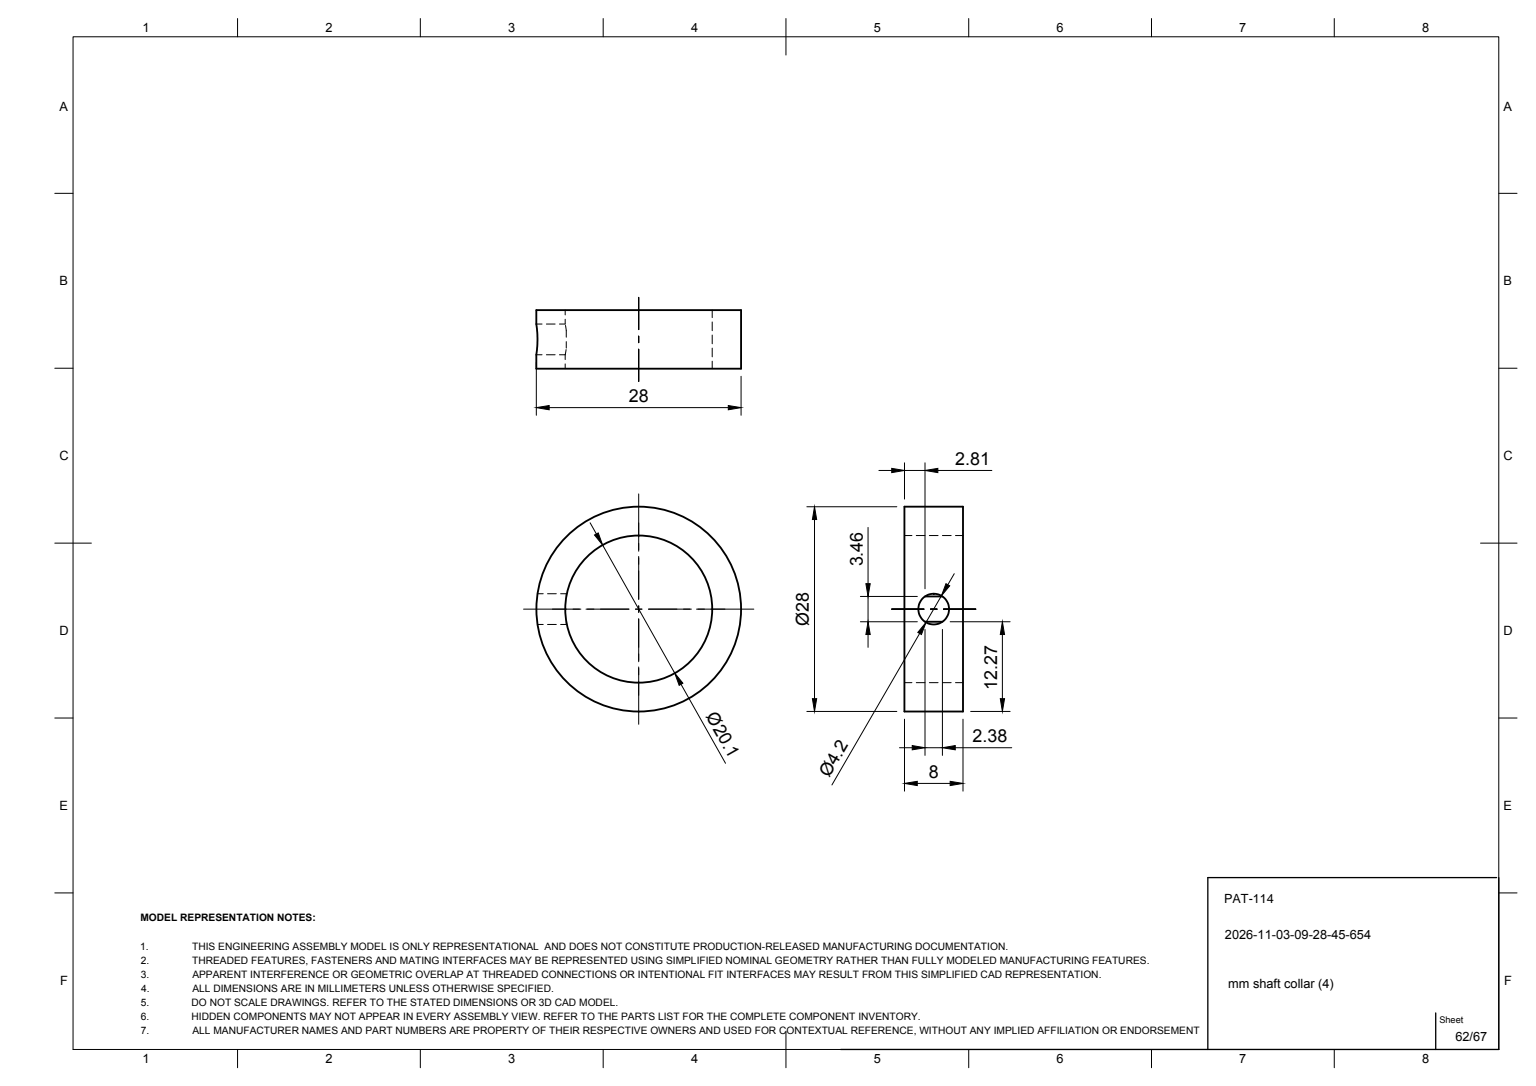
ISO-10303-21;
HEADER;
/* Generated by software containing ST-Developer
 * from STEP Tools, Inc. (www.steptools.com) 
 */

FILE_DESCRIPTION(
/* description */ ('Two-stage gear reducer in split housing'),
/* implementation_level */ '2;1');

FILE_NAME(
/* name */ 'mm shaft collar (4).step',
/* time_stamp */ '2026-10-28T03:22:31-07:00',
/* author */ (''),
/* organization */ (''),
/* preprocessor_version */ 'ST-DEVELOPER v20.2',
/* originating_system */ 'Autodesk Translation Framework v15.17.0.0',
/* authorisation */ '');

FILE_SCHEMA (('AUTOMOTIVE_DESIGN { 1 0 10303 214 3 1 1 }'));
ENDSEC;

DATA;
#10=MECHANICAL_DESIGN_GEOMETRIC_PRESENTATION_REPRESENTATION('',(#1296),#73366);
#979=B_SPLINE_CURVE_WITH_KNOTS('',3,(#49298,#49299,#49300,#49301,#49302,
#49303,#49304,#49305,#49306,#49307,#49308,#49309,#49310,#49311),
 .UNSPECIFIED.,.F.,.F.,(4,2,2,2,2,2,4),(0.756005737987022,0.79356882756465,
0.872922520054205,0.95227621254376,1.03162990503331,1.11098359752287,1.14854668710049),
 .UNSPECIFIED.);
#980=B_SPLINE_CURVE_WITH_KNOTS('',3,(#49317,#49318,#49319,#49320,#49321,
#49322,#49323,#49324,#49325,#49326,#49327,#49328,#49329,#49330,#49331,#49332,
#49333,#49334),.UNSPECIFIED.,.F.,.F.,(4,2,2,2,2,2,2,2,4),(0.,0.0792334805614376,
0.158466961122875,0.237699060165218,0.316931159207561,0.396163258249904,
0.475395357292247,0.554628837853685,0.633862318415122),.UNSPECIFIED.);
#981=B_SPLINE_CURVE_WITH_KNOTS('',3,(#49335,#49336,#49337,#49338,#49339,
#49340,#49341,#49342,#49343,#49344,#49345,#49346,#49347,#49348,#49349,#49350,
#49351,#49352),.UNSPECIFIED.,.F.,.F.,(4,2,2,2,2,2,2,2,4),(0.633862318415122,
0.71309579897656,0.792329279537998,0.871561378580341,0.950793477622684,
1.03002557666503,1.10925767570737,1.18849115626881,1.26772463683024),
 .UNSPECIFIED.);
#982=B_SPLINE_CURVE_WITH_KNOTS('',3,(#49355,#49356,#49357,#49358,#49359,
#49360,#49361,#49362,#49363,#49364,#49365,#49366,#49367,#49368),
 .UNSPECIFIED.,.F.,.F.,(4,2,2,2,2,2,4),(0.121154929624522,0.158718019202143,
0.238071711691698,0.317425404181253,0.396779096670808,0.476132789160363,
0.513695878737986),.UNSPECIFIED.);
#1169=SHAPE_REPRESENTATION_RELATIONSHIP('SRR','None',#73661,#1225);
#1225=ADVANCED_BREP_SHAPE_REPRESENTATION('',(#1365),#73357);
#1296=STYLED_ITEM('',(#73988),#1365);
#1365=MANIFOLD_SOLID_BREP('Body1',#16186);
#1582=FACE_BOUND('',#3820,.T.);
#1583=FACE_BOUND('',#3822,.T.);
#1584=FACE_BOUND('',#3824,.T.);
#1585=FACE_BOUND('',#3826,.T.);
#1921=PLANE('',#18152);
#1922=PLANE('',#18157);
#1923=PLANE('',#18164);
#1924=PLANE('',#18165);
#2695=FACE_OUTER_BOUND('',#3816,.T.);
#2696=FACE_OUTER_BOUND('',#3817,.T.);
#2697=FACE_OUTER_BOUND('',#3818,.T.);
#2698=FACE_OUTER_BOUND('',#3819,.T.);
#2699=FACE_OUTER_BOUND('',#3821,.T.);
#2700=FACE_OUTER_BOUND('',#3823,.T.);
#2701=FACE_OUTER_BOUND('',#3825,.T.);
#3816=EDGE_LOOP('',(#13707,#13708));
#3817=EDGE_LOOP('',(#13709,#13710,#13711,#13712,#13713,#13714,#13715,#13716,
#13717));
#3818=EDGE_LOOP('',(#13718,#13719,#13720));
#3819=EDGE_LOOP('',(#13721,#13722,#13723,#13724));
#3820=EDGE_LOOP('',(#13725,#13726,#13727,#13728));
#3821=EDGE_LOOP('',(#13729,#13730,#13731,#13732));
#3822=EDGE_LOOP('',(#13733,#13734));
#3823=EDGE_LOOP('',(#13735));
#3824=EDGE_LOOP('',(#13736));
#3825=EDGE_LOOP('',(#13737));
#3826=EDGE_LOOP('',(#13738));
#4846=LINE('',#49294,#5870);
#4847=LINE('',#49315,#5871);
#4848=LINE('',#49370,#5872);
#4849=LINE('',#49375,#5873);
#4850=LINE('',#49381,#5874);
#5870=VECTOR('',#21930,1.);
#5871=VECTOR('',#21937,0.210000000000001);
#5872=VECTOR('',#21942,1.);
#5873=VECTOR('',#21947,1.005);
#5874=VECTOR('',#21954,1.4);
#6706=CIRCLE('',#18153,0.210000000000001);
#6707=CIRCLE('',#18155,0.210000000000001);
#6708=CIRCLE('',#18156,0.210000000000001);
#6709=CIRCLE('',#18159,1.005);
#6710=CIRCLE('',#18160,1.005);
#6711=CIRCLE('',#18162,1.4);
#6712=CIRCLE('',#18163,1.4);
#7907=VERTEX_POINT('',#49292);
#7908=VERTEX_POINT('',#49293);
#7909=VERTEX_POINT('',#49297);
#7910=VERTEX_POINT('',#49312);
#7911=VERTEX_POINT('',#49314);
#7912=VERTEX_POINT('',#49316);
#7913=VERTEX_POINT('',#49353);
#7914=VERTEX_POINT('',#49372);
#7915=VERTEX_POINT('',#49374);
#7916=VERTEX_POINT('',#49378);
#7917=VERTEX_POINT('',#49380);
#9907=EDGE_CURVE('',#7907,#7908,#4846,.T.);
#9908=EDGE_CURVE('',#7907,#7908,#6706,.T.);
#9909=EDGE_CURVE('',#7909,#7907,#979,.T.);
#9910=EDGE_CURVE('',#7910,#7909,#6707,.T.);
#9911=EDGE_CURVE('',#7910,#7911,#4847,.T.);
#9912=EDGE_CURVE('',#7912,#7911,#980,.T.);
#9913=EDGE_CURVE('',#7911,#7912,#981,.T.);
#9914=EDGE_CURVE('',#7913,#7910,#6708,.T.);
#9915=EDGE_CURVE('',#7908,#7913,#982,.T.);
#9916=EDGE_CURVE('',#7913,#7909,#4848,.T.);
#9917=EDGE_CURVE('',#7914,#7914,#6709,.T.);
#9918=EDGE_CURVE('',#7914,#7915,#4849,.T.);
#9919=EDGE_CURVE('',#7915,#7915,#6710,.T.);
#9920=EDGE_CURVE('',#7916,#7916,#6711,.T.);
#9921=EDGE_CURVE('',#7916,#7917,#4850,.T.);
#9922=EDGE_CURVE('',#7917,#7917,#6712,.T.);
#13707=ORIENTED_EDGE('',*,*,#9907,.F.);
#13708=ORIENTED_EDGE('',*,*,#9908,.T.);
#13709=ORIENTED_EDGE('',*,*,#9909,.F.);
#13710=ORIENTED_EDGE('',*,*,#9910,.F.);
#13711=ORIENTED_EDGE('',*,*,#9911,.T.);
#13712=ORIENTED_EDGE('',*,*,#9912,.F.);
#13713=ORIENTED_EDGE('',*,*,#9913,.F.);
#13714=ORIENTED_EDGE('',*,*,#9911,.F.);
#13715=ORIENTED_EDGE('',*,*,#9914,.F.);
#13716=ORIENTED_EDGE('',*,*,#9915,.F.);
#13717=ORIENTED_EDGE('',*,*,#9908,.F.);
#13718=ORIENTED_EDGE('',*,*,#9916,.F.);
#13719=ORIENTED_EDGE('',*,*,#9914,.T.);
#13720=ORIENTED_EDGE('',*,*,#9910,.T.);
#13721=ORIENTED_EDGE('',*,*,#9917,.F.);
#13722=ORIENTED_EDGE('',*,*,#9918,.T.);
#13723=ORIENTED_EDGE('',*,*,#9919,.T.);
#13724=ORIENTED_EDGE('',*,*,#9918,.F.);
#13725=ORIENTED_EDGE('',*,*,#9915,.T.);
#13726=ORIENTED_EDGE('',*,*,#9916,.T.);
#13727=ORIENTED_EDGE('',*,*,#9909,.T.);
#13728=ORIENTED_EDGE('',*,*,#9907,.T.);
#13729=ORIENTED_EDGE('',*,*,#9920,.F.);
#13730=ORIENTED_EDGE('',*,*,#9921,.T.);
#13731=ORIENTED_EDGE('',*,*,#9922,.T.);
#13732=ORIENTED_EDGE('',*,*,#9921,.F.);
#13733=ORIENTED_EDGE('',*,*,#9912,.T.);
#13734=ORIENTED_EDGE('',*,*,#9913,.T.);
#13735=ORIENTED_EDGE('',*,*,#9920,.T.);
#13736=ORIENTED_EDGE('',*,*,#9917,.T.);
#13737=ORIENTED_EDGE('',*,*,#9922,.F.);
#13738=ORIENTED_EDGE('',*,*,#9919,.F.);
#15152=CYLINDRICAL_SURFACE('',#18154,0.210000000000001);
#15153=CYLINDRICAL_SURFACE('',#18158,1.005);
#15154=CYLINDRICAL_SURFACE('',#18161,1.4);
#15902=ADVANCED_FACE('',(#2695),#1921,.T.);
#15903=ADVANCED_FACE('',(#2696),#15152,.F.);
#15904=ADVANCED_FACE('',(#2697),#1922,.T.);
#15905=ADVANCED_FACE('',(#2698,#1582),#15153,.F.);
#15906=ADVANCED_FACE('',(#2699,#1583),#15154,.T.);
#15907=ADVANCED_FACE('',(#2700,#1584),#1923,.T.);
#15908=ADVANCED_FACE('',(#2701,#1585),#1924,.F.);
#16186=CLOSED_SHELL('',(#15902,#15903,#15904,#15905,#15906,#15907,#15908));
#18151=AXIS2_PLACEMENT_3D('',#49290,#21926,#21927);
#18152=AXIS2_PLACEMENT_3D('',#49291,#21928,#21929);
#18153=AXIS2_PLACEMENT_3D('',#49295,#21931,#21932);
#18154=AXIS2_PLACEMENT_3D('',#49296,#21933,#21934);
#18155=AXIS2_PLACEMENT_3D('',#49313,#21935,#21936);
#18156=AXIS2_PLACEMENT_3D('',#49354,#21938,#21939);
#18157=AXIS2_PLACEMENT_3D('',#49369,#21940,#21941);
#18158=AXIS2_PLACEMENT_3D('',#49371,#21943,#21944);
#18159=AXIS2_PLACEMENT_3D('',#49373,#21945,#21946);
#18160=AXIS2_PLACEMENT_3D('',#49376,#21948,#21949);
#18161=AXIS2_PLACEMENT_3D('',#49377,#21950,#21951);
#18162=AXIS2_PLACEMENT_3D('',#49379,#21952,#21953);
#18163=AXIS2_PLACEMENT_3D('',#49382,#21955,#21956);
#18164=AXIS2_PLACEMENT_3D('',#49383,#21957,#21958);
#18165=AXIS2_PLACEMENT_3D('',#49384,#21959,#21960);
#21926=DIRECTION('axis',(0.,0.,1.));
#21927=DIRECTION('refdir',(1.,0.,0.));
#21928=DIRECTION('center_axis',(0.,0.,1.));
#21929=DIRECTION('ref_axis',(1.,0.,0.));
#21930=DIRECTION('',(0.,1.,0.));
#21931=DIRECTION('center_axis',(0.,0.,1.));
#21932=DIRECTION('ref_axis',(1.,0.,0.));
#21933=DIRECTION('center_axis',(0.,0.,1.));
#21934=DIRECTION('ref_axis',(1.,0.,0.));
#21935=DIRECTION('center_axis',(0.,0.,1.));
#21936=DIRECTION('ref_axis',(1.,0.,0.));
#21937=DIRECTION('',(0.,0.,1.));
#21938=DIRECTION('center_axis',(0.,0.,1.));
#21939=DIRECTION('ref_axis',(1.,0.,0.));
#21940=DIRECTION('center_axis',(0.,0.,1.));
#21941=DIRECTION('ref_axis',(1.,0.,0.));
#21942=DIRECTION('',(0.,-1.,0.));
#21943=DIRECTION('center_axis',(0.,1.,0.));
#21944=DIRECTION('ref_axis',(1.,0.,0.));
#21945=DIRECTION('center_axis',(0.,-1.,0.));
#21946=DIRECTION('ref_axis',(1.,0.,0.));
#21947=DIRECTION('',(0.,-1.,0.));
#21948=DIRECTION('center_axis',(0.,-1.,0.));
#21949=DIRECTION('ref_axis',(1.,0.,0.));
#21950=DIRECTION('center_axis',(0.,1.,0.));
#21951=DIRECTION('ref_axis',(1.,0.,0.));
#21952=DIRECTION('center_axis',(0.,1.,0.));
#21953=DIRECTION('ref_axis',(1.,0.,0.));
#21954=DIRECTION('',(0.,-1.,0.));
#21955=DIRECTION('center_axis',(0.,1.,0.));
#21956=DIRECTION('ref_axis',(1.,0.,0.));
#21957=DIRECTION('center_axis',(0.,1.,0.));
#21958=DIRECTION('ref_axis',(1.,0.,0.));
#21959=DIRECTION('center_axis',(0.,1.,0.));
#21960=DIRECTION('ref_axis',(1.,0.,0.));
#49290=CARTESIAN_POINT('',(0.,0.,0.));
#49291=CARTESIAN_POINT('Origin',(12.,-8.2,10.99));
#49292=CARTESIAN_POINT('',(12.1729884389201,-8.31905880899792,10.99));
#49293=CARTESIAN_POINT('',(12.1729884389201,-8.08094119100208,10.99));
#49294=CARTESIAN_POINT('',(12.1729884389201,-8.6,10.99));
#49295=CARTESIAN_POINT('Origin',(12.,-8.2,10.99));
#49296=CARTESIAN_POINT('Origin',(12.,-8.2,10.99));
#49297=CARTESIAN_POINT('',(11.8270115610799,-8.31905880899792,10.99));
#49298=CARTESIAN_POINT('Ctrl Pts',(11.8270115610799,-8.31905880899792,10.99));
#49299=CARTESIAN_POINT('Ctrl Pts',(11.8344051346887,-8.3298014223953,10.9912919219764));
#49300=CARTESIAN_POINT('Ctrl Pts',(11.8427028612744,-8.33968770937274,10.992653949439));
#49301=CARTESIAN_POINT('Ctrl Pts',(11.8701079261549,-8.36709277425327,10.9967480843909));
#49302=CARTESIAN_POINT('Ctrl Pts',(11.8936698322407,-8.38324205633295,10.9996958932764));
#49303=CARTESIAN_POINT('Ctrl Pts',(11.9453870953676,-8.40469779396491,11.0038502947236));
#49304=CARTESIAN_POINT('Ctrl Pts',(11.9735487691701,-8.41,11.005));
#49305=CARTESIAN_POINT('Ctrl Pts',(12.0264512308299,-8.41,11.005));
#49306=CARTESIAN_POINT('Ctrl Pts',(12.0546129046324,-8.40469779396491,11.0038502947236));
#49307=CARTESIAN_POINT('Ctrl Pts',(12.1063301677593,-8.38324205633295,10.9996958932764));
#49308=CARTESIAN_POINT('Ctrl Pts',(12.1298920738451,-8.36709277425327,10.9967480843909));
#49309=CARTESIAN_POINT('Ctrl Pts',(12.1572971387256,-8.33968770937274,10.992653949439));
#49310=CARTESIAN_POINT('Ctrl Pts',(12.1655948653113,-8.32980142239529,10.9912919219764));
#49311=CARTESIAN_POINT('Ctrl Pts',(12.1729884389201,-8.31905880899792,10.99));
#49312=CARTESIAN_POINT('',(11.79,-8.2,10.99));
#49313=CARTESIAN_POINT('Origin',(12.,-8.2,10.99));
#49314=CARTESIAN_POINT('',(11.79,-8.2,11.38416039533));
#49315=CARTESIAN_POINT('',(11.79,-8.2,10.99));
#49316=CARTESIAN_POINT('',(12.21,-8.2,11.38416039533));
#49317=CARTESIAN_POINT('Ctrl Pts',(12.21,-8.2,11.38416039533));
#49318=CARTESIAN_POINT('Ctrl Pts',(12.21,-8.22641116018714,11.38416039533));
#49319=CARTESIAN_POINT('Ctrl Pts',(12.2047135491119,-8.2545550596171,11.3849944296993));
#49320=CARTESIAN_POINT('Ctrl Pts',(12.1832699958585,-8.30628264999174,11.3879947099895));
#49321=CARTESIAN_POINT('Ctrl Pts',(12.1671150376064,-8.32986981049192,11.3901162943626));
#49322=CARTESIAN_POINT('Ctrl Pts',(12.1298701351968,-8.36711471290156,11.394089123191));
#49323=CARTESIAN_POINT('Ctrl Pts',(12.1062828345902,-8.38326992585508,11.3962002442067));
#49324=CARTESIAN_POINT('Ctrl Pts',(12.0545547656039,-8.40471366447292,11.3991765222353));
#49325=CARTESIAN_POINT('Ctrl Pts',(12.0264106996808,-8.41,11.4));
#49326=CARTESIAN_POINT('Ctrl Pts',(11.9735893003192,-8.41,11.4));
#49327=CARTESIAN_POINT('Ctrl Pts',(11.9454452343961,-8.40471366447292,11.3991765222353));
#49328=CARTESIAN_POINT('Ctrl Pts',(11.8937171654098,-8.38326992585508,11.3962002442067));
#49329=CARTESIAN_POINT('Ctrl Pts',(11.8701298648032,-8.36711471290156,11.394089123191));
#49330=CARTESIAN_POINT('Ctrl Pts',(11.8328849623936,-8.32986981049192,11.3901162943626));
#49331=CARTESIAN_POINT('Ctrl Pts',(11.8167300041415,-8.30628264999174,11.3879947099895));
#49332=CARTESIAN_POINT('Ctrl Pts',(11.7952864508881,-8.2545550596171,11.3849944296993));
#49333=CARTESIAN_POINT('Ctrl Pts',(11.79,-8.22641116018714,11.38416039533));
#49334=CARTESIAN_POINT('Ctrl Pts',(11.79,-8.2,11.38416039533));
#49335=CARTESIAN_POINT('Ctrl Pts',(11.79,-8.2,11.38416039533));
#49336=CARTESIAN_POINT('Ctrl Pts',(11.79,-8.17358883981285,11.38416039533));
#49337=CARTESIAN_POINT('Ctrl Pts',(11.7952864508881,-8.1454449403829,11.3849944296993));
#49338=CARTESIAN_POINT('Ctrl Pts',(11.8167300041415,-8.09371735000826,11.3879947099895));
#49339=CARTESIAN_POINT('Ctrl Pts',(11.8328849623936,-8.07013018950807,11.3901162943626));
#49340=CARTESIAN_POINT('Ctrl Pts',(11.8701298648032,-8.03288528709843,11.394089123191));
#49341=CARTESIAN_POINT('Ctrl Pts',(11.8937171654098,-8.01673007414492,11.3962002442067));
#49342=CARTESIAN_POINT('Ctrl Pts',(11.9454452343961,-7.99528633552708,11.3991765222353));
#49343=CARTESIAN_POINT('Ctrl Pts',(11.9735893003192,-7.99,11.4));
#49344=CARTESIAN_POINT('Ctrl Pts',(12.0264106996808,-7.99,11.4));
#49345=CARTESIAN_POINT('Ctrl Pts',(12.0545547656039,-7.99528633552708,11.3991765222353));
#49346=CARTESIAN_POINT('Ctrl Pts',(12.1062828345902,-8.01673007414492,11.3962002442067));
#49347=CARTESIAN_POINT('Ctrl Pts',(12.1298701351968,-8.03288528709843,11.394089123191));
#49348=CARTESIAN_POINT('Ctrl Pts',(12.1671150376064,-8.07013018950807,11.3901162943626));
#49349=CARTESIAN_POINT('Ctrl Pts',(12.1832699958585,-8.09371735000826,11.3879947099895));
#49350=CARTESIAN_POINT('Ctrl Pts',(12.2047135491119,-8.1454449403829,11.3849944296993));
#49351=CARTESIAN_POINT('Ctrl Pts',(12.21,-8.17358883981285,11.38416039533));
#49352=CARTESIAN_POINT('Ctrl Pts',(12.21,-8.2,11.38416039533));
#49353=CARTESIAN_POINT('',(11.8270115610799,-8.08094119100208,10.99));
#49354=CARTESIAN_POINT('Origin',(12.,-8.2,10.99));
#49355=CARTESIAN_POINT('Ctrl Pts',(12.1729884389201,-8.08094119100208,10.99));
#49356=CARTESIAN_POINT('Ctrl Pts',(12.1655948653113,-8.07019857760471,10.9912919219764));
#49357=CARTESIAN_POINT('Ctrl Pts',(12.1572971387256,-8.06031229062725,10.992653949439));
#49358=CARTESIAN_POINT('Ctrl Pts',(12.1298920738451,-8.03290722574673,10.9967480843909));
#49359=CARTESIAN_POINT('Ctrl Pts',(12.1063301677593,-8.01675794366705,10.9996958932764));
#49360=CARTESIAN_POINT('Ctrl Pts',(12.0546129046324,-7.99530220603509,11.0038502947236));
#49361=CARTESIAN_POINT('Ctrl Pts',(12.0264512308299,-7.99,11.005));
#49362=CARTESIAN_POINT('Ctrl Pts',(11.9735487691701,-7.99,11.005));
#49363=CARTESIAN_POINT('Ctrl Pts',(11.9453870953676,-7.99530220603509,11.0038502947236));
#49364=CARTESIAN_POINT('Ctrl Pts',(11.8936698322407,-8.01675794366705,10.9996958932764));
#49365=CARTESIAN_POINT('Ctrl Pts',(11.8701079261549,-8.03290722574673,10.9967480843909));
#49366=CARTESIAN_POINT('Ctrl Pts',(11.8427028612744,-8.06031229062725,10.992653949439));
#49367=CARTESIAN_POINT('Ctrl Pts',(11.8344051346887,-8.0701985776047,10.9912919219764));
#49368=CARTESIAN_POINT('Ctrl Pts',(11.8270115610799,-8.08094119100208,10.99));
#49369=CARTESIAN_POINT('Origin',(12.,-8.2,10.99));
#49370=CARTESIAN_POINT('',(11.8270115610799,-8.6,10.99));
#49371=CARTESIAN_POINT('Origin',(12.,-8.6,10.));
#49372=CARTESIAN_POINT('',(10.995,-7.8,10.));
#49373=CARTESIAN_POINT('Origin',(12.,-7.8,10.));
#49374=CARTESIAN_POINT('',(10.995,-8.6,10.));
#49375=CARTESIAN_POINT('',(10.995,-8.6,10.));
#49376=CARTESIAN_POINT('Origin',(12.,-8.6,10.));
#49377=CARTESIAN_POINT('Origin',(12.,-8.6,10.));
#49378=CARTESIAN_POINT('',(10.6,-7.8,10.));
#49379=CARTESIAN_POINT('Origin',(12.,-7.8,10.));
#49380=CARTESIAN_POINT('',(10.6,-8.6,10.));
#49381=CARTESIAN_POINT('',(10.6,-8.6,10.));
#49382=CARTESIAN_POINT('Origin',(12.,-8.6,10.));
#49383=CARTESIAN_POINT('Origin',(12.,-7.8,10.));
#49384=CARTESIAN_POINT('Origin',(12.,-8.6,10.));
#73293=UNCERTAINTY_MEASURE_WITH_UNIT(LENGTH_MEASURE(0.001),#73367,
'DISTANCE_ACCURACY_VALUE',
'Maximum model space distance between geometric entities at asserted c
onnectivities');
#73302=UNCERTAINTY_MEASURE_WITH_UNIT(LENGTH_MEASURE(0.001),#73367,
'DISTANCE_ACCURACY_VALUE',
'Maximum model space distance between geometric entities at asserted c
onnectivities');
#73357=(
GEOMETRIC_REPRESENTATION_CONTEXT(3)
GLOBAL_UNCERTAINTY_ASSIGNED_CONTEXT((#73293))
GLOBAL_UNIT_ASSIGNED_CONTEXT((#73367,#73369,#73370))
REPRESENTATION_CONTEXT('','3D')
);
#73366=(
GEOMETRIC_REPRESENTATION_CONTEXT(3)
GLOBAL_UNCERTAINTY_ASSIGNED_CONTEXT((#73302))
GLOBAL_UNIT_ASSIGNED_CONTEXT((#73367,#73369,#73370))
REPRESENTATION_CONTEXT('','3D')
);
#73367=(
LENGTH_UNIT()
NAMED_UNIT(*)
SI_UNIT(.CENTI.,.METRE.)
);
#73369=(
NAMED_UNIT(*)
PLANE_ANGLE_UNIT()
SI_UNIT($,.RADIAN.)
);
#73370=(
NAMED_UNIT(*)
SI_UNIT($,.STERADIAN.)
SOLID_ANGLE_UNIT()
);
#73425=SHAPE_DEFINITION_REPRESENTATION(#73558,#73661);
#73558=PRODUCT_DEFINITION_SHAPE('',$,#73725);
#73661=SHAPE_REPRESENTATION('',(#18151),#73357);
#73670=PRODUCT_DEFINITION_CONTEXT('part definition',#73861,'design');
#73725=PRODUCT_DEFINITION('mm shaft collar (4)','mm shaft collar (4)',#73788,
#73670);
#73788=PRODUCT_DEFINITION_FORMATION('',$,#73917);
#73861=APPLICATION_CONTEXT(
'Core Data for Automotive Mechanical Design Process');
#73862=PRODUCT_CONTEXT('part definition',#73861,'mechanical');
#73917=PRODUCT('mm shaft collar (4)','mm shaft collar (4)',
'mm shaft collar (4)',(#73862));
#73982=COLOUR_RGB('Grey',0.48,0.52,0.57);
#73983=FILL_AREA_STYLE_COLOUR('',#73982);
#73984=FILL_AREA_STYLE('',(#73983));
#73985=SURFACE_STYLE_FILL_AREA(#73984);
#73986=SURFACE_SIDE_STYLE('',(#73985));
#73987=SURFACE_STYLE_USAGE(.BOTH.,#73986);
#73988=PRESENTATION_STYLE_ASSIGNMENT((#73987));
ENDSEC;
END-ISO-10303-21;
